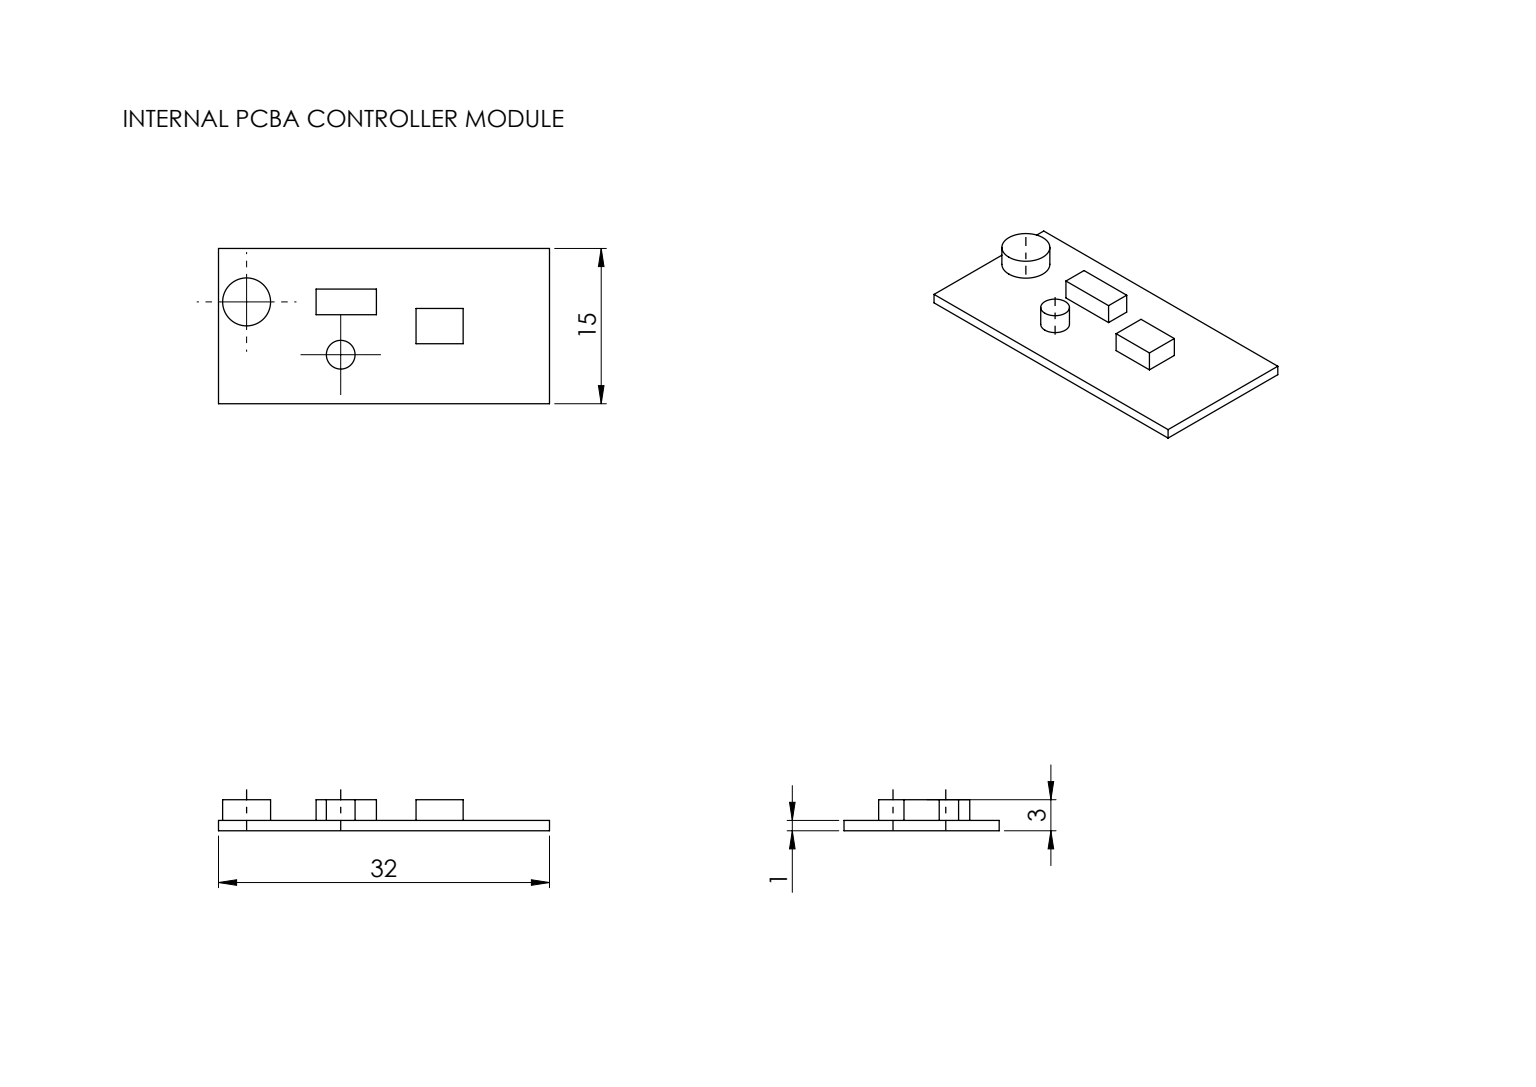
ISO-10303-21;
HEADER;
FILE_DESCRIPTION (('STEP AP214'),
    '1' );
FILE_NAME ('Internal PCBA Controller Module.step',
    '2026-10-02T09:26:43',
    ( '' ),
    ( '' ),
    'SwSTEP 2.0',
    'SolidWorks 2026',
    '' );
FILE_SCHEMA (( 'AUTOMOTIVE_DESIGN' ));
ENDSEC;

DATA;
#61=CARTESIAN_POINT ( 'NONE',  ( 139.9358549477330200, 0.5000000000000000000, -1.098523788719517169 ) ) ;
#111=CARTESIAN_POINT ( 'NONE',  ( 133.2169897921533845, 2.500000000000000000, -4.655597831175330548 ) ) ;
#208=FILL_AREA_STYLE ('',( #102307 ) ) ;
#396=PLANE ( 'NONE',  #56788 ) ;
#491=VECTOR ( 'NONE', #65782, 1000.000000000000000 ) ;
#598=DIRECTION ( 'NONE',  ( 0.000000000000000000, 0.000000000000000000, -1.000000000000000000 ) ) ;
#785=AXIS2_PLACEMENT_3D ( 'NONE', #25187, #6184, #3623 ) ;
#1353=DIRECTION ( 'NONE',  ( 1.000000000000000000, 0.000000000000000000, 0.000000000000000000 ) ) ;
#1618=AXIS2_PLACEMENT_3D ( 'NONE', #115980, #104231, #44031 ) ;
#1686=AXIS2_PLACEMENT_3D ( 'NONE', #69594, #89239, #129198 ) ;
#1783=ADVANCED_FACE ( 'NONE', ( #63659 ), #47886, .F. ) ;
#1952=LINE ( 'NONE', #55582, #72543 ) ;
#1992=EDGE_LOOP ( 'NONE', ( #83331, #6563, #5558, #78744 ) ) ;
#2013=VECTOR ( 'NONE', #33725, 1000.000000000000000 ) ;
#2082=CARTESIAN_POINT ( 'NONE',  ( 0.000000000000000000, 2.500000000000000000, 0.000000000000000000 ) ) ;
#2160=DIRECTION ( 'NONE',  ( 1.000000000000000000, 0.000000000000000000, 0.000000000000000000 ) ) ;
#2750=ORIENTED_EDGE ( 'NONE', *, *, #14810, .F. ) ;
#2868=VERTEX_POINT ( 'NONE', #9576 ) ;
#3123=FACE_BOUND ( 'NONE', #89319, .T. ) ;
#3196=DIRECTION ( 'NONE',  ( -0.000000000000000000, -1.000000000000000000, -0.000000000000000000 ) ) ;
#3623=DIRECTION ( 'NONE',  ( 0.000000000000000000, -0.000000000000000000, 1.000000000000000000 ) ) ;
#3643=ORIENTED_EDGE ( 'NONE', *, *, #119168, .T. ) ;
#3721=EDGE_LOOP ( 'NONE', ( #14930, #97877, #94219, #80001 ) ) ;
#3749=ADVANCED_FACE ( 'NONE', ( #85573 ), #33279, .F. ) ;
#4146=ORIENTED_EDGE ( 'NONE', *, *, #13081, .F. ) ;
#4176=VERTEX_POINT ( 'NONE', #110095 ) ;
#4584=DIRECTION ( 'NONE',  ( 0.000000000000000000, -0.000000000000000000, 1.000000000000000000 ) ) ;
#4890=CARTESIAN_POINT ( 'NONE',  ( 149.5981739382431783, 2.500000000000000000, 1.703575533167231537 ) ) ;
#5071=DIRECTION ( 'NONE',  ( 1.000000000000000000, 0.000000000000000000, -1.084202172485504434E-16 ) ) ;
#5285=CARTESIAN_POINT ( 'NONE',  ( 139.9358549477330200, 2.500000000000000000, -3.576063159858998475 ) ) ;
#5558=ORIENTED_EDGE ( 'NONE', *, *, #35698, .F. ) ;
#5707=CARTESIAN_POINT ( 'NONE',  ( 154.1524742528378056, 0.5000000000000000000, 1.703575533167231537 ) ) ;
#5990=SURFACE_SIDE_STYLE ('',( #85210 ) ) ;
#6007=CARTESIAN_POINT ( 'NONE',  ( 130.5000000000000000, -0.5000000000000000000, 7.499999999999998224 ) ) ;
#6184=DIRECTION ( 'NONE',  ( 0.000000000000000000, 1.000000000000000000, 0.000000000000000000 ) ) ;
#6305=AXIS2_PLACEMENT_3D ( 'NONE', #84477, #104735, #4584 ) ;
#6563=ORIENTED_EDGE ( 'NONE', *, *, #82060, .F. ) ;
#6883=EDGE_CURVE ( 'NONE', #54857, #102205, #70700, .T. ) ;
#6965=EDGE_LOOP ( 'NONE', ( #83440, #68214, #37688, #13118 ) ) ;
#7061=EDGE_LOOP ( 'NONE', ( #21290, #56050 ) ) ;
#7353=AXIS2_PLACEMENT_3D ( 'NONE', #115499, #75583, #67039 ) ;
#7874=FACE_OUTER_BOUND ( 'NONE', #93186, .T. ) ;
#8253=ORIENTED_EDGE ( 'NONE', *, *, #14810, .T. ) ;
#8378=AXIS2_PLACEMENT_3D ( 'NONE', #66138, #106073, #107999 ) ;
#8513=CARTESIAN_POINT ( 'NONE',  ( 162.5000000000000000, -0.5000000000000000000, -7.500000000000005329 ) ) ;
#9576=CARTESIAN_POINT ( 'NONE',  ( 142.3152275665817115, 0.5000000000000000000, 4.152444035927816302 ) ) ;
#9599=DIRECTION ( 'NONE',  ( -1.000000000000000000, -0.000000000000000000, -0.000000000000000000 ) ) ;
#9893=LINE ( 'NONE', #61, #77548 ) ;
#9916=AXIS2_PLACEMENT_3D ( 'NONE', #78615, #38022, #77944 ) ;
#9974=VECTOR ( 'NONE', #56454, 1000.000000000000000 ) ;
#10039=CARTESIAN_POINT ( 'NONE',  ( 162.5000000000000000, 0.5000000000000000000, -7.500000000000005329 ) ) ;
#10059=LINE ( 'NONE', #110195, #83855 ) ;
#10241=FACE_OUTER_BOUND ( 'NONE', #80105, .T. ) ;
#10407=ORIENTED_EDGE ( 'NONE', *, *, #13081, .T. ) ;
#10478=ORIENTED_EDGE ( 'NONE', *, *, #61124, .T. ) ;
#10519=EDGE_LOOP ( 'NONE', ( #14019, #2750, #22603, #90684 ) ) ;
#10639=VERTEX_POINT ( 'NONE', #6007 ) ;
#10644=CARTESIAN_POINT ( 'NONE',  ( 0.000000000000000000, 0.000000000000000000, 0.000000000000000000 ) ) ;
#10757=VECTOR ( 'NONE', #106512, 1000.000000000000000 ) ;
#10957=ORIENTED_EDGE ( 'NONE', *, *, #27576, .T. ) ;
#11366=CARTESIAN_POINT ( 'NONE',  ( 162.5000000000000000, 0.5000000000000000000, -7.500000000000005329 ) ) ;
#11835=CARTESIAN_POINT ( 'NONE',  ( 139.9358549477330200, 2.500000000000000000, -3.576063159858998475 ) ) ;
#11990=VERTEX_POINT ( 'NONE', #40618 ) ;
#12151=AXIS2_PLACEMENT_3D ( 'NONE', #80067, #19864, #119995 ) ;
#12406=ORIENTED_EDGE ( 'NONE', *, *, #65701, .T. ) ;
#12503=PLANE ( 'NONE',  #85742 ) ;
#12613=SURFACE_SIDE_STYLE ('',( #121939 ) ) ;
#12975=CARTESIAN_POINT ( 'NONE',  ( 142.3152275665817115, 2.500000000000000000, 4.152444035927816302 ) ) ;
#13081=EDGE_CURVE ( 'NONE', #86648, #112541, #57109, .T. ) ;
#13118=ORIENTED_EDGE ( 'NONE', *, *, #102486, .T. ) ;
#13186=DIRECTION ( 'NONE',  ( 0.000000000000000000, -0.000000000000000000, 1.000000000000000000 ) ) ;
#13431=VECTOR ( 'NONE', #66560, 1000.000000000000000 ) ;
#13502=CARTESIAN_POINT ( 'NONE',  ( 145.7653593504141725, 0.5000000000000000000, -3.576063159858998475 ) ) ;
#13560=AXIS2_PLACEMENT_3D ( 'NONE', #118011, #28360, #95800 ) ;
#13601=PLANE ( 'NONE',  #20802 ) ;
#13681=ORIENTED_EDGE ( 'NONE', *, *, #25639, .T. ) ;
#13709=DIRECTION ( 'NONE',  ( 0.000000000000000000, 0.000000000000000000, 1.000000000000000000 ) ) ;
#13884=SURFACE_STYLE_USAGE ( .BOTH. , #5990 ) ;
#13959=ORIENTED_EDGE ( 'NONE', *, *, #40890, .T. ) ;
#14019=ORIENTED_EDGE ( 'NONE', *, *, #43973, .T. ) ;
#14045=UNCERTAINTY_MEASURE_WITH_UNIT (LENGTH_MEASURE( 1.000000000000000082E-05 ), #22472, 'distance_accuracy_value', 'NONE');
#14204=DIRECTION ( 'NONE',  ( 0.000000000000000000, 1.000000000000000000, 0.000000000000000000 ) ) ;
#14467=CARTESIAN_POINT ( 'NONE',  ( 133.2169897921533845, 0.5000000000000000000, -0.01898911740318533561 ) ) ;
#14810=EDGE_CURVE ( 'NONE', #34747, #62008, #64855, .T. ) ;
#14860=DIRECTION ( 'NONE',  ( 0.000000000000000000, 0.000000000000000000, 1.000000000000000000 ) ) ;
#14930=ORIENTED_EDGE ( 'NONE', *, *, #99140, .F. ) ;
#15162=MECHANICAL_DESIGN_GEOMETRIC_PRESENTATION_REPRESENTATION('',(#56927),#17210);
#15699=EDGE_CURVE ( 'NONE', #104225, #83642, #112378, .T. ) ;
#16019=ADVANCED_FACE ( 'NONE', ( #91766 ), #92401, .T. ) ;
#16201=EDGE_LOOP ( 'NONE', ( #89223, #108455, #3643, #45452 ) ) ;
#16389=DIRECTION ( 'NONE',  ( -0.000000000000000000, -0.000000000000000000, -1.000000000000000000 ) ) ;
#16519=CARTESIAN_POINT ( 'NONE',  ( 133.2169897921533845, 2.500000000000000000, -4.655597831175330548 ) ) ;
#16562=LINE ( 'NONE', #104324, #48735 ) ;
#16982=CARTESIAN_POINT ( 'NONE',  ( 154.1524742528378056, 2.500000000000000000, -1.703575533167231537 ) ) ;
#17147=DIRECTION ( 'NONE',  ( -0.000000000000000000, -1.000000000000000000, -0.000000000000000000 ) ) ;
#17210=( GEOMETRIC_REPRESENTATION_CONTEXT ( 3 ) GLOBAL_UNCERTAINTY_ASSIGNED_CONTEXT ( ( #14045 ) ) GLOBAL_UNIT_ASSIGNED_CONTEXT ( ( #22472, #129212, #51921 ) ) REPRESENTATION_CONTEXT ( 'NONE', 'WORKASPACE' ) );
#17798=CARTESIAN_POINT ( 'NONE',  ( 149.5981739382431783, 0.5000000000000000000, -1.703575533167231537 ) ) ;
#17924=APPLICATION_CONTEXT ( 'automotive_design' ) ;
#18114=DIRECTION ( 'NONE',  ( 0.000000000000000000, 0.000000000000000000, -1.000000000000000000 ) ) ;
#18288=EDGE_CURVE ( 'NONE', #70042, #49008, #44429, .T. ) ;
#18424=VECTOR ( 'NONE', #41452, 1000.000000000000000 ) ;
#19326=ORIENTED_EDGE ( 'NONE', *, *, #40152, .F. ) ;
#19545=PLANE ( 'NONE',  #115654 ) ;
#19570=CARTESIAN_POINT ( 'NONE',  ( 149.5981739382431783, 2.500000000000000000, 1.703575533167231537 ) ) ;
#19670=ORIENTED_EDGE ( 'NONE', *, *, #40152, .T. ) ;
#19864=DIRECTION ( 'NONE',  ( -0.000000000000000000, -1.000000000000000000, -0.000000000000000000 ) ) ;
#19875=EDGE_CURVE ( 'NONE', #37705, #4176, #75349, .T. ) ;
#20589=ADVANCED_FACE ( 'NONE', ( #86567 ), #57111, .T. ) ;
#20689=CARTESIAN_POINT ( 'NONE',  ( 130.5000000000000000, 0.5000000000000000000, 7.499999999999998224 ) ) ;
#20802=AXIS2_PLACEMENT_3D ( 'NONE', #25349, #65927, #45666 ) ;
#20814=CARTESIAN_POINT ( 'NONE',  ( 162.5000000000000000, -0.5000000000000000000, 7.499999999999994671 ) ) ;
#21137=FACE_OUTER_BOUND ( 'NONE', #70487, .T. ) ;
#21244=CARTESIAN_POINT ( 'NONE',  ( 133.2169897921533845, 2.500000000000000000, -2.337293474289257933 ) ) ;
#21290=ORIENTED_EDGE ( 'NONE', *, *, #30432, .T. ) ;
#21819=SURFACE_STYLE_USAGE ( .BOTH. , #12613 ) ;
#22472=( LENGTH_UNIT ( ) NAMED_UNIT ( * ) SI_UNIT ( .MILLI., .METRE. ) );
#22564=ADVANCED_FACE ( 'NONE', ( #109202 ), #19545, .F. ) ;
#22603=ORIENTED_EDGE ( 'NONE', *, *, #65701, .F. ) ;
#23083=EDGE_CURVE ( 'NONE', #4176, #10639, #30528, .T. ) ;
#23103=EDGE_LOOP ( 'NONE', ( #36300, #59458 ) ) ;
#23423=DIRECTION ( 'NONE',  ( 1.084202172485504434E-16, -0.000000000000000000, 1.000000000000000000 ) ) ;
#23907=VECTOR ( 'NONE', #113347, 1000.000000000000000 ) ;
#24055=EDGE_LOOP ( 'NONE', ( #40407, #101634, #105706, #26760 ) ) ;
#24276=ADVANCED_FACE ( 'NONE', ( #10241 ), #396, .F. ) ;
#24693=DIRECTION ( 'NONE',  ( 0.000000000000000000, 0.000000000000000000, 1.000000000000000000 ) ) ;
#25029=CARTESIAN_POINT ( 'NONE',  ( 133.2169897921533845, 0.5000000000000000000, -4.655597831175330548 ) ) ;
#25187=CARTESIAN_POINT ( 'NONE',  ( 133.2169897921533845, 2.500000000000000000, -2.337293474289257933 ) ) ;
#25349=CARTESIAN_POINT ( 'NONE',  ( 139.9358549477330200, 2.500000000000000000, -3.576063159858998475 ) ) ;
#25358=AXIS2_PLACEMENT_3D ( 'NONE', #125675, #49091, #598 ) ;
#25639=EDGE_CURVE ( 'NONE', #44247, #77073, #59607, .T. ) ;
#26495=EDGE_CURVE ( 'NONE', #117877, #112541, #89210, .T. ) ;
#26601=LINE ( 'NONE', #66508, #87205 ) ;
#26760=ORIENTED_EDGE ( 'NONE', *, *, #92525, .T. ) ;
#26825=DIRECTION ( 'NONE',  ( 0.000000000000000000, -0.000000000000000000, 1.000000000000000000 ) ) ;
#26933=ORIENTED_EDGE ( 'NONE', *, *, #107201, .F. ) ;
#26948=DIRECTION ( 'NONE',  ( -1.000000000000000000, 0.000000000000000000, -0.000000000000000000 ) ) ;
#27283=CARTESIAN_POINT ( 'NONE',  ( 149.5981739382431783, 0.5000000000000000000, 1.703575533167231537 ) ) ;
#27500=DIRECTION ( 'NONE',  ( -0.000000000000000000, -1.000000000000000000, -0.000000000000000000 ) ) ;
#27576=EDGE_CURVE ( 'NONE', #86599, #110722, #33227, .T. ) ;
#28107=ORIENTED_EDGE ( 'NONE', *, *, #120172, .T. ) ;
#28360=DIRECTION ( 'NONE',  ( 0.000000000000000000, 1.000000000000000000, 0.000000000000000000 ) ) ;
#28585=CARTESIAN_POINT ( 'NONE',  ( 149.5981739382431783, 2.500000000000000000, -1.703575533167231537 ) ) ;
#28690=VERTEX_POINT ( 'NONE', #77802 ) ;
#29807=DIRECTION ( 'NONE',  ( 0.000000000000000000, 0.000000000000000000, -1.000000000000000000 ) ) ;
#29930=VECTOR ( 'NONE', #73992, 1000.000000000000000 ) ;
#30207=ORIENTED_EDGE ( 'NONE', *, *, #40786, .F. ) ;
#30325=EDGE_LOOP ( 'NONE', ( #77414, #45887, #65344, #115571 ) ) ;
#30432=EDGE_CURVE ( 'NONE', #86599, #28690, #57484, .T. ) ;
#30528=LINE ( 'NONE', #20689, #36456 ) ;
#30686=EDGE_LOOP ( 'NONE', ( #63549, #119398, #71516, #120626 ) ) ;
#31267=LINE ( 'NONE', #62658, #109837 ) ;
#31683=ORIENTED_EDGE ( 'NONE', *, *, #15699, .F. ) ;
#32674=AXIS2_PLACEMENT_3D ( 'NONE', #63607, #104169, #74707 ) ;
#32686=AXIS2_PLACEMENT_3D ( 'NONE', #33242, #82977, #92124 ) ;
#32743=PLANE ( 'NONE',  #40256 ) ;
#32771=DIRECTION ( 'NONE',  ( -0.000000000000000000, -0.000000000000000000, -1.000000000000000000 ) ) ;
#33184=EDGE_CURVE ( 'NONE', #50067, #54857, #10059, .T. ) ;
#33227=LINE ( 'NONE', #73132, #113990 ) ;
#33242=CARTESIAN_POINT ( 'NONE',  ( 0.000000000000000000, 0.5000000000000000000, 0.000000000000000000 ) ) ;
#33279=PLANE ( 'NONE',  #54019 ) ;
#33446=ADVANCED_FACE ( 'NONE', ( #115195 ), #45850, .F. ) ;
#33725=DIRECTION ( 'NONE',  ( 1.000000000000000000, 0.000000000000000000, 0.000000000000000000 ) ) ;
#33856=FACE_BOUND ( 'NONE', #23103, .T. ) ;
#33922=ORIENTED_EDGE ( 'NONE', *, *, #100074, .F. ) ;
#34197=( NAMED_UNIT ( * ) SI_UNIT ( $, .STERADIAN. ) SOLID_ANGLE_UNIT ( ) );
#34567=CARTESIAN_POINT ( 'NONE',  ( 162.5000000000000000, 0.5000000000000000000, -7.500000000000005329 ) ) ;
#34673=ORIENTED_EDGE ( 'NONE', *, *, #35638, .T. ) ;
#34747=VERTEX_POINT ( 'NONE', #113159 ) ;
#35072=ORIENTED_EDGE ( 'NONE', *, *, #107639, .F. ) ;
#35319=DIRECTION ( 'NONE',  ( 1.000000000000000000, -0.000000000000000000, -1.084202172485504434E-16 ) ) ;
#35388=AXIS2_PLACEMENT_3D ( 'NONE', #11366, #98444, #38931 ) ;
#35483=FILL_AREA_STYLE ('',( #66208 ) ) ;
#35638=EDGE_CURVE ( 'NONE', #70042, #119203, #86366, .T. ) ;
#35698=EDGE_CURVE ( 'NONE', #4176, #104225, #16562, .T. ) ;
#36203=CARTESIAN_POINT ( 'NONE',  ( 0.000000000000000000, -0.5000000000000000000, 0.000000000000000000 ) ) ;
#36216=AXIS2_PLACEMENT_3D ( 'NONE', #21244, #71642, #72931 ) ;
#36253=ORIENTED_EDGE ( 'NONE', *, *, #107201, .T. ) ;
#36300=ORIENTED_EDGE ( 'NONE', *, *, #61124, .F. ) ;
#36456=VECTOR ( 'NONE', #112293, 1000.000000000000000 ) ;
#36596=ORIENTED_EDGE ( 'NONE', *, *, #6883, .T. ) ;
#36663=PLANE ( 'NONE',  #77580 ) ;
#36815=ORIENTED_EDGE ( 'NONE', *, *, #116805, .T. ) ;
#37667=EDGE_LOOP ( 'NONE', ( #50089, #99755, #58404, #85578 ) ) ;
#37688=ORIENTED_EDGE ( 'NONE', *, *, #72322, .F. ) ;
#37705=VERTEX_POINT ( 'NONE', #101594 ) ;
#37972=FACE_OUTER_BOUND ( 'NONE', #16201, .T. ) ;
#38022=DIRECTION ( 'NONE',  ( 0.000000000000000000, 0.000000000000000000, -1.000000000000000000 ) ) ;
#38442=LINE ( 'NONE', #108438, #10757 ) ;
#38571=DIRECTION ( 'NONE',  ( -1.000000000000000000, 0.000000000000000000, 1.084202172485504434E-16 ) ) ;
#38931=DIRECTION ( 'NONE',  ( 0.000000000000000000, 0.000000000000000000, 1.000000000000000000 ) ) ;
#39634=EDGE_CURVE ( 'NONE', #83642, #37705, #1952, .T. ) ;
#39846=VERTEX_POINT ( 'NONE', #20814 ) ;
#40130=ADVANCED_FACE ( 'NONE', ( #21137 ), #120634, .T. ) ;
#40152=EDGE_CURVE ( 'NONE', #83642, #44247, #48678, .T. ) ;
#40242=EDGE_CURVE ( 'NONE', #2868, #110722, #58145, .T. ) ;
#40256=AXIS2_PLACEMENT_3D ( 'NONE', #51729, #13709, #101469 ) ;
#40287=ORIENTED_EDGE ( 'NONE', *, *, #114150, .T. ) ;
#40407=ORIENTED_EDGE ( 'NONE', *, *, #40786, .T. ) ;
#40618=CARTESIAN_POINT ( 'NONE',  ( 145.7653593504141725, 0.5000000000000000000, -3.576063159858998475 ) ) ;
#40626=CARTESIAN_POINT ( 'NONE',  ( 145.7653593504141725, 2.500000000000000000, -1.098523788719517169 ) ) ;
#40786=EDGE_CURVE ( 'NONE', #88966, #44639, #123061, .T. ) ;
#40890=EDGE_CURVE ( 'NONE', #124382, #117877, #56238, .T. ) ;
#40988=AXIS2_PLACEMENT_3D ( 'NONE', #106716, #27500, #125702 ) ;
#41452=DIRECTION ( 'NONE',  ( -0.000000000000000000, -1.000000000000000000, -0.000000000000000000 ) ) ;
#41855=CARTESIAN_POINT ( 'NONE',  ( 154.1524742528378056, 2.500000000000000000, 1.703575533167231537 ) ) ;
#42492=ORIENTED_EDGE ( 'NONE', *, *, #95835, .T. ) ;
#43073=PLANE ( 'NONE',  #32686 ) ;
#43181=VECTOR ( 'NONE', #74376, 1000.000000000000000 ) ;
#43237=VECTOR ( 'NONE', #69116, 1000.000000000000000 ) ;
#43499=CIRCLE ( 'NONE', #129200, 2.318304356886072615 ) ;
#43573=( GEOMETRIC_REPRESENTATION_CONTEXT ( 3 ) GLOBAL_UNCERTAINTY_ASSIGNED_CONTEXT ( ( #121523 ) ) GLOBAL_UNIT_ASSIGNED_CONTEXT ( ( #115286, #55749, #95689 ) ) REPRESENTATION_CONTEXT ( 'NONE', 'WORKASPACE' ) );
#43973=EDGE_CURVE ( 'NONE', #11990, #62008, #31267, .T. ) ;
#44015=( NAMED_UNIT ( * ) PLANE_ANGLE_UNIT ( ) SI_UNIT ( $, .RADIAN. ) );
#44031=DIRECTION ( 'NONE',  ( 0.000000000000000000, 0.000000000000000000, 1.000000000000000000 ) ) ;
#44169=FACE_OUTER_BOUND ( 'NONE', #116361, .T. ) ;
#44247=VERTEX_POINT ( 'NONE', #76336 ) ;
#44320=FACE_BOUND ( 'NONE', #30325, .T. ) ;
#44429=LINE ( 'NONE', #122999, #52762 ) ;
#44639=VERTEX_POINT ( 'NONE', #105480 ) ;
#44777=VECTOR ( 'NONE', #89682, 1000.000000000000000 ) ;
#45235=DIRECTION ( 'NONE',  ( -0.000000000000000000, -1.000000000000000000, -0.000000000000000000 ) ) ;
#45452=ORIENTED_EDGE ( 'NONE', *, *, #56592, .T. ) ;
#45454=EDGE_CURVE ( 'NONE', #37705, #77073, #26601, .T. ) ;
#45571=CARTESIAN_POINT ( 'NONE',  ( 149.5981739382431783, 2.500000000000000000, -1.703575533167231537 ) ) ;
#45666=DIRECTION ( 'NONE',  ( 0.000000000000000000, 0.000000000000000000, -1.000000000000000000 ) ) ;
#45850=PLANE ( 'NONE',  #25358 ) ;
#45887=ORIENTED_EDGE ( 'NONE', *, *, #121541, .F. ) ;
#46473=CARTESIAN_POINT ( 'NONE',  ( 149.5981739382431783, 0.5000000000000000000, 1.703575533167231537 ) ) ;
#46543=FACE_OUTER_BOUND ( 'NONE', #118945, .T. ) ;
#47036=CIRCLE ( 'NONE', #13560, 2.318304356886072615 ) ;
#47302=CARTESIAN_POINT ( 'NONE',  ( 149.5981739382431783, 2.500000000000000000, 1.703575533167231537 ) ) ;
#47791=ORIENTED_EDGE ( 'NONE', *, *, #67874, .F. ) ;
#47886=PLANE ( 'NONE',  #72691 ) ;
#48273=ORIENTED_EDGE ( 'NONE', *, *, #76882, .F. ) ;
#48395=ORIENTED_EDGE ( 'NONE', *, *, #56592, .F. ) ;
#48678=LINE ( 'NONE', #10039, #18424 ) ;
#48735=VECTOR ( 'NONE', #96415, 1000.000000000000000 ) ;
#49008=VERTEX_POINT ( 'NONE', #14467 ) ;
#49033=VERTEX_POINT ( 'NONE', #127515 ) ;
#49091=DIRECTION ( 'NONE',  ( 1.000000000000000000, 0.000000000000000000, 0.000000000000000000 ) ) ;
#49246=EDGE_LOOP ( 'NONE', ( #86440, #127359, #110430, #94128 ) ) ;
#49560=ORIENTED_EDGE ( 'NONE', *, *, #86041, .F. ) ;
#49832=COLOUR_RGB ( '', 0.31764706, 0.68627451, 0.89019608) ;
#49841=CARTESIAN_POINT ( 'NONE',  ( 162.5000000000000000, 0.5000000000000000000, 7.499999999999994671 ) ) ;
#50067=VERTEX_POINT ( 'NONE', #90481 ) ;
#50089=ORIENTED_EDGE ( 'NONE', *, *, #19875, .T. ) ;
#51459=ORIENTED_EDGE ( 'NONE', *, *, #56230, .F. ) ;
#51729=CARTESIAN_POINT ( 'NONE',  ( 149.5981739382431783, 2.500000000000000000, -1.703575533167231537 ) ) ;
#51890=VECTOR ( 'NONE', #17147, 1000.000000000000000 ) ;
#51921=( NAMED_UNIT ( * ) SI_UNIT ( $, .STERADIAN. ) SOLID_ANGLE_UNIT ( ) );
#52159=UNCERTAINTY_MEASURE_WITH_UNIT (LENGTH_MEASURE( 1.000000000000000082E-05 ), #103580, 'distance_accuracy_value', 'NONE');
#52762=VECTOR ( 'NONE', #102697, 1000.000000000000000 ) ;
#53084=DIRECTION ( 'NONE',  ( 0.000000000000000000, 0.000000000000000000, 1.000000000000000000 ) ) ;
#54019=AXIS2_PLACEMENT_3D ( 'NONE', #34567, #23423, #5071 ) ;
#54819=ORIENTED_EDGE ( 'NONE', *, *, #25639, .F. ) ;
#54857=VERTEX_POINT ( 'NONE', #74561 ) ;
#55281=ORIENTED_EDGE ( 'NONE', *, *, #26495, .F. ) ;
#55335=CARTESIAN_POINT ( 'NONE',  ( 154.1524742528378056, 2.500000000000000000, -1.703575533167231537 ) ) ;
#55424=AXIS2_PLACEMENT_3D ( 'NONE', #104256, #76086, #56430 ) ;
#55582=CARTESIAN_POINT ( 'NONE',  ( 162.5000000000000000, 0.5000000000000000000, -7.500000000000005329 ) ) ;
#55658=DIRECTION ( 'NONE',  ( -0.000000000000000000, -1.000000000000000000, -0.000000000000000000 ) ) ;
#55746=LINE ( 'NONE', #57022, #77152 ) ;
#55749=( NAMED_UNIT ( * ) PLANE_ANGLE_UNIT ( ) SI_UNIT ( $, .RADIAN. ) );
#55757=AXIS2_PLACEMENT_3D ( 'NONE', #96944, #116581, #57684 ) ;
#55901=PRODUCT_DEFINITION_CONTEXT ( 'detailed design', #83124, 'design' ) ;
#55938=DIRECTION ( 'NONE',  ( -0.000000000000000000, -1.000000000000000000, -0.000000000000000000 ) ) ;
#56050=ORIENTED_EDGE ( 'NONE', *, *, #99140, .T. ) ;
#56230=EDGE_CURVE ( 'NONE', #10639, #39846, #123661, .T. ) ;
#56238=LINE ( 'NONE', #126284, #56942 ) ;
#56430=DIRECTION ( 'NONE',  ( 0.000000000000000000, 0.000000000000000000, 1.000000000000000000 ) ) ;
#56454=DIRECTION ( 'NONE',  ( -0.000000000000000000, -1.000000000000000000, -0.000000000000000000 ) ) ;
#56460=DIRECTION ( 'NONE',  ( 0.000000000000000000, -0.000000000000000000, -1.000000000000000000 ) ) ;
#56546=ORIENTED_EDGE ( 'NONE', *, *, #6883, .F. ) ;
#56592=EDGE_CURVE ( 'NONE', #99284, #49008, #43499, .T. ) ;
#56788=AXIS2_PLACEMENT_3D ( 'NONE', #99916, #110368, #18114 ) ;
#56864=PRODUCT_CONTEXT ( 'NONE', #17924, 'mechanical' ) ;
#56927=STYLED_ITEM ( 'NONE', ( #60465 ), #57280 ) ;
#56942=VECTOR ( 'NONE', #57543, 1000.000000000000000 ) ;
#57022=CARTESIAN_POINT ( 'NONE',  ( 145.7653593504141725, 2.500000000000000000, -3.576063159858998475 ) ) ;
#57109=LINE ( 'NONE', #47302, #51890 ) ;
#57111=PLANE ( 'NONE',  #123787 ) ;
#57280=MANIFOLD_SOLID_BREP ( 'Boss-Extrude2', #89605 ) ;
#57484=CIRCLE ( 'NONE', #55424, 1.388921157871087386 ) ;
#57543=DIRECTION ( 'NONE',  ( -0.000000000000000000, -1.000000000000000000, -0.000000000000000000 ) ) ;
#57548=EDGE_LOOP ( 'NONE', ( #33922, #54819, #26933, #51459 ) ) ;
#57684=DIRECTION ( 'NONE',  ( 1.000000000000000000, 0.000000000000000000, -0.000000000000000000 ) ) ;
#57948=ORIENTED_EDGE ( 'NONE', *, *, #26495, .T. ) ;
#58145=CIRCLE ( 'NONE', #1686, 1.388921157871087386 ) ;
#58233=DIRECTION ( 'NONE',  ( 0.000000000000000000, 1.000000000000000000, 0.000000000000000000 ) ) ;
#58307=ADVANCED_FACE ( 'NONE', ( #114851 ), #114226, .T. ) ;
#58404=ORIENTED_EDGE ( 'NONE', *, *, #15699, .T. ) ;
#58989=DIRECTION ( 'NONE',  ( 0.000000000000000000, 0.000000000000000000, -1.000000000000000000 ) ) ;
#59138=ORIENTED_EDGE ( 'NONE', *, *, #121057, .T. ) ;
#59458=ORIENTED_EDGE ( 'NONE', *, *, #40242, .F. ) ;
#59607=LINE ( 'NONE', #117174, #44777 ) ;
#60143=DIRECTION ( 'NONE',  ( -1.084202172485504434E-16, 0.000000000000000000, -1.000000000000000000 ) ) ;
#60465=PRESENTATION_STYLE_ASSIGNMENT (( #21819 ) ) ;
#60833=EDGE_LOOP ( 'NONE', ( #99588, #34673 ) ) ;
#61124=EDGE_CURVE ( 'NONE', #110722, #2868, #89086, .T. ) ;
#61369=ORIENTED_EDGE ( 'NONE', *, *, #33184, .F. ) ;
#61627=FACE_OUTER_BOUND ( 'NONE', #24055, .T. ) ;
#62008=VERTEX_POINT ( 'NONE', #72962 ) ;
#62280=CIRCLE ( 'NONE', #1618, 1.388921157871087386 ) ;
#62658=CARTESIAN_POINT ( 'NONE',  ( 139.9358549477330200, 0.5000000000000000000, -3.576063159858998475 ) ) ;
#63166=VECTOR ( 'NONE', #92728, 1000.000000000000000 ) ;
#63549=ORIENTED_EDGE ( 'NONE', *, *, #93014, .T. ) ;
#63573=CARTESIAN_POINT ( 'NONE',  ( 145.7653593504141725, 2.500000000000000000, -3.576063159858998475 ) ) ;
#63607=CARTESIAN_POINT ( 'NONE',  ( 142.3152275665817115, 0.5000000000000000000, 2.763522878056728693 ) ) ;
#63659=FACE_OUTER_BOUND ( 'NONE', #119127, .T. ) ;
#64518=VECTOR ( 'NONE', #55938, 1000.000000000000000 ) ;
#64634=LINE ( 'NONE', #104562, #83491 ) ;
#64855=LINE ( 'NONE', #5285, #124731 ) ;
#65273=VECTOR ( 'NONE', #32771, 1000.000000000000000 ) ;
#65344=ORIENTED_EDGE ( 'NONE', *, *, #121057, .F. ) ;
#65701=EDGE_CURVE ( 'NONE', #49033, #34747, #81861, .T. ) ;
#65736=DIRECTION ( 'NONE',  ( -1.000000000000000000, 0.000000000000000000, 0.000000000000000000 ) ) ;
#65782=DIRECTION ( 'NONE',  ( -0.000000000000000000, -0.000000000000000000, -1.000000000000000000 ) ) ;
#65890=CARTESIAN_POINT ( 'NONE',  ( 133.2169897921533845, 0.5000000000000000000, -2.337293474289257933 ) ) ;
#65927=DIRECTION ( 'NONE',  ( 1.000000000000000000, 0.000000000000000000, 0.000000000000000000 ) ) ;
#66038=DIRECTION ( 'NONE',  ( -1.000000000000000000, 0.000000000000000000, 1.084202172485504434E-16 ) ) ;
#66138=CARTESIAN_POINT ( 'NONE',  ( 133.2169897921533845, 2.500000000000000000, -2.337293474289257933 ) ) ;
#66208=FILL_AREA_STYLE_COLOUR ( '', #49832 ) ;
#66387=CARTESIAN_POINT ( 'NONE',  ( 145.7653593504141725, 2.500000000000000000, -3.576063159858998475 ) ) ;
#66508=CARTESIAN_POINT ( 'NONE',  ( 130.5000000000000000, 0.5000000000000000000, -7.500000000000001776 ) ) ;
#66523=STYLED_ITEM ( 'NONE', ( #95044 ), #122749 ) ;
#66560=DIRECTION ( 'NONE',  ( 1.000000000000000000, 0.000000000000000000, 0.000000000000000000 ) ) ;
#67039=DIRECTION ( 'NONE',  ( 0.000000000000000000, 0.000000000000000000, 1.000000000000000000 ) ) ;
#67874=EDGE_CURVE ( 'NONE', #124382, #86648, #117571, .T. ) ;
#68022=VECTOR ( 'NONE', #109498, 1000.000000000000000 ) ;
#68214=ORIENTED_EDGE ( 'NONE', *, *, #40890, .F. ) ;
#69116=DIRECTION ( 'NONE',  ( 0.000000000000000000, 0.000000000000000000, 1.000000000000000000 ) ) ;
#69449=DIRECTION ( 'NONE',  ( -0.000000000000000000, -1.000000000000000000, -0.000000000000000000 ) ) ;
#69594=CARTESIAN_POINT ( 'NONE',  ( 142.3152275665817115, 0.5000000000000000000, 2.763522878056728693 ) ) ;
#69644=PLANE ( 'NONE',  #35388 ) ;
#70042=VERTEX_POINT ( 'NONE', #92350 ) ;
#70487=EDGE_LOOP ( 'NONE', ( #78003, #123559, #42492, #73890 ) ) ;
#70700=LINE ( 'NONE', #40626, #86914 ) ;
#70895=ORIENTED_EDGE ( 'NONE', *, *, #30432, .F. ) ;
#71516=ORIENTED_EDGE ( 'NONE', *, *, #67874, .T. ) ;
#71642=DIRECTION ( 'NONE',  ( 0.000000000000000000, 1.000000000000000000, 0.000000000000000000 ) ) ;
#72322=EDGE_CURVE ( 'NONE', #129134, #124382, #74699, .T. ) ;
#72543=VECTOR ( 'NONE', #66038, 1000.000000000000000 ) ;
#72691=AXIS2_PLACEMENT_3D ( 'NONE', #127089, #58989, #26948 ) ;
#72765=DIRECTION ( 'NONE',  ( -1.000000000000000000, -0.000000000000000000, -0.000000000000000000 ) ) ;
#72931=DIRECTION ( 'NONE',  ( 0.000000000000000000, 0.000000000000000000, 1.000000000000000000 ) ) ;
#72962=CARTESIAN_POINT ( 'NONE',  ( 139.9358549477330200, 0.5000000000000000000, -3.576063159858998475 ) ) ;
#73132=CARTESIAN_POINT ( 'NONE',  ( 142.3152275665817115, 2.500000000000000000, 1.374601720185641973 ) ) ;
#73890=ORIENTED_EDGE ( 'NONE', *, *, #119168, .F. ) ;
#73992=DIRECTION ( 'NONE',  ( -1.000000000000000000, -0.000000000000000000, -0.000000000000000000 ) ) ;
#74254=AXIS2_PLACEMENT_3D ( 'NONE', #89375, #119456, #29807 ) ;
#74376=DIRECTION ( 'NONE',  ( -0.000000000000000000, -0.000000000000000000, -1.000000000000000000 ) ) ;
#74561=CARTESIAN_POINT ( 'NONE',  ( 145.7653593504141725, 2.500000000000000000, -1.098523788719517169 ) ) ;
#74699=LINE ( 'NONE', #113325, #108637 ) ;
#74707=DIRECTION ( 'NONE',  ( 0.000000000000000000, 0.000000000000000000, 1.000000000000000000 ) ) ;
#75349=LINE ( 'NONE', #106110, #23907 ) ;
#75574=CARTESIAN_POINT ( 'NONE',  ( 139.9358549477330200, 2.500000000000000000, -1.098523788719517169 ) ) ;
#75583=DIRECTION ( 'NONE',  ( 0.000000000000000000, 1.000000000000000000, 0.000000000000000000 ) ) ;
#75737=VECTOR ( 'NONE', #83835, 1000.000000000000000 ) ;
#76043=SHAPE_REPRESENTATION_RELATIONSHIP ( 'NONE' , 'NONE' ,  #125483, #122749 ) ;
#76086=DIRECTION ( 'NONE',  ( 0.000000000000000000, 1.000000000000000000, 0.000000000000000000 ) ) ;
#76336=CARTESIAN_POINT ( 'NONE',  ( 162.5000000000000000, -0.5000000000000000000, -7.500000000000005329 ) ) ;
#76522=ADVANCED_FACE ( 'NONE', ( #61627 ), #12503, .F. ) ;
#76530=ORIENTED_EDGE ( 'NONE', *, *, #86293, .F. ) ;
#76587=FACE_OUTER_BOUND ( 'NONE', #30686, .T. ) ;
#76625=ADVANCED_FACE ( 'NONE', ( #76587 ), #95587, .T. ) ;
#76882=EDGE_CURVE ( 'NONE', #28690, #2868, #81730, .T. ) ;
#77073=VERTEX_POINT ( 'NONE', #96065 ) ;
#77152=VECTOR ( 'NONE', #126435, 1000.000000000000000 ) ;
#77175=SHAPE_DEFINITION_REPRESENTATION ( #87007, #125483 ) ;
#77414=ORIENTED_EDGE ( 'NONE', *, *, #114150, .F. ) ;
#77548=VECTOR ( 'NONE', #1353, 1000.000000000000000 ) ;
#77580=AXIS2_PLACEMENT_3D ( 'NONE', #116474, #58233, #26825 ) ;
#77694=PRODUCT_DEFINITION_FORMATION_WITH_SPECIFIED_SOURCE ( 'ANY', '', #95331, .NOT_KNOWN. ) ;
#77802=CARTESIAN_POINT ( 'NONE',  ( 142.3152275665817115, 2.500000000000000000, 4.152444035927816302 ) ) ;
#77824=EDGE_CURVE ( 'NONE', #49033, #11990, #99791, .T. ) ;
#77944=DIRECTION ( 'NONE',  ( -1.000000000000000000, 0.000000000000000000, -0.000000000000000000 ) ) ;
#78003=ORIENTED_EDGE ( 'NONE', *, *, #35638, .F. ) ;
#78111=CARTESIAN_POINT ( 'NONE',  ( 149.5981739382431783, 0.5000000000000000000, -1.703575533167231537 ) ) ;
#78279=FACE_OUTER_BOUND ( 'NONE', #3721, .T. ) ;
#78325=LINE ( 'NONE', #129367, #100454 ) ;
#78615=CARTESIAN_POINT ( 'NONE',  ( 139.9358549477330200, 2.500000000000000000, -1.098523788719517169 ) ) ;
#78744=ORIENTED_EDGE ( 'NONE', *, *, #23083, .T. ) ;
#79265=ORIENTED_EDGE ( 'NONE', *, *, #120172, .F. ) ;
#79592=LINE ( 'NONE', #98555, #43237 ) ;
#80001=ORIENTED_EDGE ( 'NONE', *, *, #27576, .F. ) ;
#80067=CARTESIAN_POINT ( 'NONE',  ( 133.2169897921533845, 2.500000000000000000, -2.337293474289257933 ) ) ;
#80105=EDGE_LOOP ( 'NONE', ( #57948, #4146, #47791, #13959 ) ) ;
#80157=EDGE_LOOP ( 'NONE', ( #48395, #89825 ) ) ;
#80365=DIRECTION ( 'NONE',  ( -1.000000000000000000, -0.000000000000000000, -0.000000000000000000 ) ) ;
#80718=DIRECTION ( 'NONE',  ( 1.000000000000000000, 0.000000000000000000, 0.000000000000000000 ) ) ;
#81668=FACE_OUTER_BOUND ( 'NONE', #37667, .T. ) ;
#81730=LINE ( 'NONE', #12975, #96295 ) ;
#81861=LINE ( 'NONE', #11835, #29930 ) ;
#81876=DIRECTION ( 'NONE',  ( -1.000000000000000000, 0.000000000000000000, 0.000000000000000000 ) ) ;
#81932=DIRECTION ( 'NONE',  ( 0.000000000000000000, 1.000000000000000000, 0.000000000000000000 ) ) ;
#82060=EDGE_CURVE ( 'NONE', #104225, #39846, #96988, .T. ) ;
#82977=DIRECTION ( 'NONE',  ( 0.000000000000000000, -1.000000000000000000, 0.000000000000000000 ) ) ;
#83041=ORIENTED_EDGE ( 'NONE', *, *, #92525, .F. ) ;
#83124=APPLICATION_CONTEXT ( 'automotive_design' ) ;
#83181=MECHANICAL_DESIGN_GEOMETRIC_PRESENTATION_REPRESENTATION('',(#66523),#43573);
#83331=ORIENTED_EDGE ( 'NONE', *, *, #56230, .T. ) ;
#83440=ORIENTED_EDGE ( 'NONE', *, *, #107639, .T. ) ;
#83491=VECTOR ( 'NONE', #14860, 1000.000000000000000 ) ;
#83636=ADVANCED_FACE ( 'NONE', ( #117205 ), #118518, .F. ) ;
#83642=VERTEX_POINT ( 'NONE', #98234 ) ;
#83835=DIRECTION ( 'NONE',  ( -0.000000000000000000, -1.000000000000000000, -0.000000000000000000 ) ) ;
#83855=VECTOR ( 'NONE', #2160, 1000.000000000000000 ) ;
#83951=VECTOR ( 'NONE', #9599, 1000.000000000000000 ) ;
#84477=CARTESIAN_POINT ( 'NONE',  ( 0.000000000000000000, 2.500000000000000000, 0.000000000000000000 ) ) ;
#85036=ORIENTED_EDGE ( 'NONE', *, *, #86293, .T. ) ;
#85210=SURFACE_STYLE_FILL_AREA ( #35483 ) ;
#85573=FACE_OUTER_BOUND ( 'NONE', #98567, .T. ) ;
#85578=ORIENTED_EDGE ( 'NONE', *, *, #39634, .T. ) ;
#85742=AXIS2_PLACEMENT_3D ( 'NONE', #123730, #81876, #53084 ) ;
#86041=EDGE_CURVE ( 'NONE', #86648, #110490, #92645, .T. ) ;
#86293=EDGE_CURVE ( 'NONE', #50067, #120204, #116145, .T. ) ;
#86366=CIRCLE ( 'NONE', #36216, 2.318304356886072615 ) ;
#86374=FACE_OUTER_BOUND ( 'NONE', #7061, .T. ) ;
#86440=ORIENTED_EDGE ( 'NONE', *, *, #100074, .T. ) ;
#86561=LINE ( 'NONE', #16519, #9974 ) ;
#86567=FACE_OUTER_BOUND ( 'NONE', #57548, .T. ) ;
#86599=VERTEX_POINT ( 'NONE', #115162 ) ;
#86648=VERTEX_POINT ( 'NONE', #19570 ) ;
#86914=VECTOR ( 'NONE', #99533, 1000.000000000000000 ) ;
#86949=ADVANCED_FACE ( 'NONE', ( #103295 ), #13601, .F. ) ;
#87007=PRODUCT_DEFINITION_SHAPE ( 'NONE', 'NONE',  #92424 ) ;
#87205=VECTOR ( 'NONE', #106442, 1000.000000000000000 ) ;
#88416=CARTESIAN_POINT ( 'NONE',  ( 139.9358549477330200, 0.5000000000000000000, -1.098523788719517169 ) ) ;
#88966=VERTEX_POINT ( 'NONE', #5707 ) ;
#89086=CIRCLE ( 'NONE', #32674, 1.388921157871087386 ) ;
#89210=LINE ( 'NONE', #78111, #68022 ) ;
#89223=ORIENTED_EDGE ( 'NONE', *, *, #18288, .F. ) ;
#89239=DIRECTION ( 'NONE',  ( 0.000000000000000000, 1.000000000000000000, 0.000000000000000000 ) ) ;
#89319=EDGE_LOOP ( 'NONE', ( #30207, #125882, #55281, #35072 ) ) ;
#89373=AXIS2_PLACEMENT_3D ( 'NONE', #66387, #65736, #106315 ) ;
#89375=CARTESIAN_POINT ( 'NONE',  ( 142.3152275665817115, 2.500000000000000000, 2.763522878056728693 ) ) ;
#89587=ADVANCED_FACE ( 'NONE', ( #89921 ), #69644, .F. ) ;
#89605=CLOSED_SHELL ( 'NONE', ( #40130, #128218, #98175, #33446, #22564, #89587, #3749, #20589, #98751, #83636, #86949, #129142, #16019, #111605, #92078, #113651, #58307, #76522, #126752, #24276, #1783, #76625 ) ) ;
#89682=DIRECTION ( 'NONE',  ( -1.000000000000000000, 0.000000000000000000, 1.084202172485504434E-16 ) ) ;
#89825=ORIENTED_EDGE ( 'NONE', *, *, #95835, .F. ) ;
#89921=FACE_OUTER_BOUND ( 'NONE', #91344, .T. ) ;
#90481=CARTESIAN_POINT ( 'NONE',  ( 139.9358549477330200, 2.500000000000000000, -1.098523788719517169 ) ) ;
#90516=DIRECTION ( 'NONE',  ( 0.000000000000000000, 0.000000000000000000, 1.000000000000000000 ) ) ;
#90684=ORIENTED_EDGE ( 'NONE', *, *, #77824, .T. ) ;
#91344=EDGE_LOOP ( 'NONE', ( #36253, #19326, #31683, #125416 ) ) ;
#91640=FACE_OUTER_BOUND ( 'NONE', #6965, .T. ) ;
#91766=FACE_OUTER_BOUND ( 'NONE', #120854, .T. ) ;
#92025=LINE ( 'NONE', #120842, #83951 ) ;
#92078=ADVANCED_FACE ( 'NONE', ( #86374 ), #36663, .T. ) ;
#92124=DIRECTION ( 'NONE',  ( 0.000000000000000000, -0.000000000000000000, -1.000000000000000000 ) ) ;
#92350=CARTESIAN_POINT ( 'NONE',  ( 133.2169897921533845, 2.500000000000000000, -0.01898911740318533561 ) ) ;
#92401=PLANE ( 'NONE',  #129051 ) ;
#92424=PRODUCT_DEFINITION ( 'UNKNOWN', '', #77694, #55901 ) ;
#92525=EDGE_CURVE ( 'NONE', #110490, #88966, #38442, .T. ) ;
#92645=LINE ( 'NONE', #4890, #2013 ) ;
#92728=DIRECTION ( 'NONE',  ( -0.000000000000000000, -0.000000000000000000, -1.000000000000000000 ) ) ;
#92877=VECTOR ( 'NONE', #69449, 1000.000000000000000 ) ;
#93014=EDGE_CURVE ( 'NONE', #110490, #129134, #125354, .T. ) ;
#93186=EDGE_LOOP ( 'NONE', ( #48273, #70895, #10957, #10478 ) ) ;
#93371=LINE ( 'NONE', #13502, #63166 ) ;
#94128=ORIENTED_EDGE ( 'NONE', *, *, #45454, .T. ) ;
#94219=ORIENTED_EDGE ( 'NONE', *, *, #40242, .T. ) ;
#94275=ORIENTED_EDGE ( 'NONE', *, *, #98526, .T. ) ;
#95044=PRESENTATION_STYLE_ASSIGNMENT (( #13884 ) ) ;
#95331=PRODUCT ( 'Internal PCBA Controller Module', 'Internal PCBA Controller Module', '', ( #56864 ) ) ;
#95587=PLANE ( 'NONE',  #6305 ) ;
#95625=CYLINDRICAL_SURFACE ( 'NONE', #40988, 1.388921157871086942 ) ;
#95689=( NAMED_UNIT ( * ) SI_UNIT ( $, .STERADIAN. ) SOLID_ANGLE_UNIT ( ) );
#95800=DIRECTION ( 'NONE',  ( 0.000000000000000000, 0.000000000000000000, 1.000000000000000000 ) ) ;
#95835=EDGE_CURVE ( 'NONE', #49008, #99284, #47036, .T. ) ;
#96065=CARTESIAN_POINT ( 'NONE',  ( 130.5000000000000000, -0.5000000000000000000, -7.500000000000001776 ) ) ;
#96134=ORIENTED_EDGE ( 'NONE', *, *, #77824, .F. ) ;
#96234=CYLINDRICAL_SURFACE ( 'NONE', #8378, 2.318304356886073059 ) ;
#96295=VECTOR ( 'NONE', #3196, 1000.000000000000000 ) ;
#96415=DIRECTION ( 'NONE',  ( 1.000000000000000000, -0.000000000000000000, -1.084202172485504434E-16 ) ) ;
#96722=CARTESIAN_POINT ( 'NONE',  ( 142.3152275665817115, 0.5000000000000000000, 1.374601720185641973 ) ) ;
#96944=CARTESIAN_POINT ( 'NONE',  ( 139.9358549477330200, 2.500000000000000000, -3.576063159858998475 ) ) ;
#96988=LINE ( 'NONE', #49841, #92877 ) ;
#97877=ORIENTED_EDGE ( 'NONE', *, *, #76882, .T. ) ;
#98175=ADVANCED_FACE ( 'NONE', ( #123518, #33856, #44320, #81668, #3123 ), #43073, .F. ) ;
#98234=CARTESIAN_POINT ( 'NONE',  ( 162.5000000000000000, 0.5000000000000000000, -7.500000000000005329 ) ) ;
#98444=DIRECTION ( 'NONE',  ( -1.000000000000000000, 0.000000000000000000, 0.000000000000000000 ) ) ;
#98526=EDGE_CURVE ( 'NONE', #34747, #50067, #79592, .T. ) ;
#98555=CARTESIAN_POINT ( 'NONE',  ( 139.9358549477330200, 2.500000000000000000, -3.576063159858998475 ) ) ;
#98561=DIRECTION ( 'NONE',  ( 0.000000000000000000, 0.000000000000000000, 1.000000000000000000 ) ) ;
#98567=EDGE_LOOP ( 'NONE', ( #13681, #114723, #121173, #19670 ) ) ;
#98751=ADVANCED_FACE ( 'NONE', ( #44169 ), #115460, .F. ) ;
#99140=EDGE_CURVE ( 'NONE', #28690, #86599, #62280, .T. ) ;
#99284=VERTEX_POINT ( 'NONE', #25029 ) ;
#99533=DIRECTION ( 'NONE',  ( -0.000000000000000000, -1.000000000000000000, -0.000000000000000000 ) ) ;
#99588=ORIENTED_EDGE ( 'NONE', *, *, #117257, .T. ) ;
#99755=ORIENTED_EDGE ( 'NONE', *, *, #35698, .T. ) ;
#99791=LINE ( 'NONE', #63573, #75737 ) ;
#99916=CARTESIAN_POINT ( 'NONE',  ( 149.5981739382431783, 2.500000000000000000, -1.703575533167231537 ) ) ;
#100074=EDGE_CURVE ( 'NONE', #77073, #10639, #64634, .T. ) ;
#100454=VECTOR ( 'NONE', #98561, 1000.000000000000000 ) ;
#101469=DIRECTION ( 'NONE',  ( 1.000000000000000000, 0.000000000000000000, -0.000000000000000000 ) ) ;
#101594=CARTESIAN_POINT ( 'NONE',  ( 130.5000000000000000, 0.5000000000000000000, -7.500000000000001776 ) ) ;
#101634=ORIENTED_EDGE ( 'NONE', *, *, #102486, .F. ) ;
#102205=VERTEX_POINT ( 'NONE', #113285 ) ;
#102307=FILL_AREA_STYLE_COLOUR ( '', #102920 ) ;
#102486=EDGE_CURVE ( 'NONE', #129134, #44639, #126344, .T. ) ;
#102697=DIRECTION ( 'NONE',  ( -0.000000000000000000, -1.000000000000000000, -0.000000000000000000 ) ) ;
#102920=COLOUR_RGB ( '', 0.31764706, 0.68627451, 0.89019608) ;
#103295=FACE_OUTER_BOUND ( 'NONE', #114993, .T. ) ;
#103512=ORIENTED_EDGE ( 'NONE', *, *, #98526, .F. ) ;
#103580=( LENGTH_UNIT ( ) NAMED_UNIT ( * ) SI_UNIT ( .MILLI., .METRE. ) );
#104169=DIRECTION ( 'NONE',  ( 0.000000000000000000, 1.000000000000000000, 0.000000000000000000 ) ) ;
#104225=VERTEX_POINT ( 'NONE', #120382 ) ;
#104231=DIRECTION ( 'NONE',  ( 0.000000000000000000, 1.000000000000000000, 0.000000000000000000 ) ) ;
#104256=CARTESIAN_POINT ( 'NONE',  ( 142.3152275665817115, 2.500000000000000000, 2.763522878056728693 ) ) ;
#104324=CARTESIAN_POINT ( 'NONE',  ( 162.5000000000000000, 0.5000000000000000000, 7.499999999999994671 ) ) ;
#104562=CARTESIAN_POINT ( 'NONE',  ( 130.5000000000000000, -0.5000000000000000000, -7.500000000000001776 ) ) ;
#104735=DIRECTION ( 'NONE',  ( 0.000000000000000000, 1.000000000000000000, 0.000000000000000000 ) ) ;
#105065=VECTOR ( 'NONE', #16389, 1000.000000000000000 ) ;
#105480=CARTESIAN_POINT ( 'NONE',  ( 154.1524742528378056, 0.5000000000000000000, -1.703575533167231537 ) ) ;
#105706=ORIENTED_EDGE ( 'NONE', *, *, #93014, .F. ) ;
#106073=DIRECTION ( 'NONE',  ( -0.000000000000000000, -1.000000000000000000, -0.000000000000000000 ) ) ;
#106092=LINE ( 'NONE', #8513, #105065 ) ;
#106110=CARTESIAN_POINT ( 'NONE',  ( 130.5000000000000000, 0.5000000000000000000, -7.500000000000001776 ) ) ;
#106243=( GEOMETRIC_REPRESENTATION_CONTEXT ( 3 ) GLOBAL_UNCERTAINTY_ASSIGNED_CONTEXT ( ( #52159 ) ) GLOBAL_UNIT_ASSIGNED_CONTEXT ( ( #103580, #44015, #34197 ) ) REPRESENTATION_CONTEXT ( 'NONE', 'WORKASPACE' ) );
#106315=DIRECTION ( 'NONE',  ( 0.000000000000000000, 0.000000000000000000, 1.000000000000000000 ) ) ;
#106442=DIRECTION ( 'NONE',  ( -0.000000000000000000, -1.000000000000000000, -0.000000000000000000 ) ) ;
#106512=DIRECTION ( 'NONE',  ( -0.000000000000000000, -1.000000000000000000, -0.000000000000000000 ) ) ;
#106716=CARTESIAN_POINT ( 'NONE',  ( 142.3152275665817115, 2.500000000000000000, 2.763522878056728693 ) ) ;
#107123=DIRECTION ( 'NONE',  ( 0.000000000000000000, 0.000000000000000000, 1.000000000000000000 ) ) ;
#107201=EDGE_CURVE ( 'NONE', #39846, #44247, #106092, .T. ) ;
#107639=EDGE_CURVE ( 'NONE', #44639, #117877, #92025, .T. ) ;
#107999=DIRECTION ( 'NONE',  ( 0.000000000000000000, 0.000000000000000000, -1.000000000000000000 ) ) ;
#108296=AXIS2_PLACEMENT_3D ( 'NONE', #10644, #90516, #80718 ) ;
#108438=CARTESIAN_POINT ( 'NONE',  ( 154.1524742528378056, 2.500000000000000000, 1.703575533167231537 ) ) ;
#108455=ORIENTED_EDGE ( 'NONE', *, *, #117257, .F. ) ;
#108637=VECTOR ( 'NONE', #72765, 1000.000000000000000 ) ;
#109202=FACE_OUTER_BOUND ( 'NONE', #1992, .T. ) ;
#109498=DIRECTION ( 'NONE',  ( 0.000000000000000000, 0.000000000000000000, 1.000000000000000000 ) ) ;
#109837=VECTOR ( 'NONE', #80365, 1000.000000000000000 ) ;
#110095=CARTESIAN_POINT ( 'NONE',  ( 130.5000000000000000, 0.5000000000000000000, 7.499999999999998224 ) ) ;
#110195=CARTESIAN_POINT ( 'NONE',  ( 139.9358549477330200, 2.500000000000000000, -1.098523788719517169 ) ) ;
#110368=DIRECTION ( 'NONE',  ( 1.000000000000000000, 0.000000000000000000, 0.000000000000000000 ) ) ;
#110430=ORIENTED_EDGE ( 'NONE', *, *, #19875, .F. ) ;
#110490=VERTEX_POINT ( 'NONE', #41855 ) ;
#110722=VERTEX_POINT ( 'NONE', #96722 ) ;
#111605=ADVANCED_FACE ( 'NONE', ( #7874 ), #95625, .T. ) ;
#111839=CIRCLE ( 'NONE', #7353, 2.318304356886072615 ) ;
#112293=DIRECTION ( 'NONE',  ( -0.000000000000000000, -1.000000000000000000, -0.000000000000000000 ) ) ;
#112378=LINE ( 'NONE', #114929, #43181 ) ;
#112541=VERTEX_POINT ( 'NONE', #46473 ) ;
#113046=DIRECTION ( 'NONE',  ( -0.000000000000000000, -1.000000000000000000, -0.000000000000000000 ) ) ;
#113159=CARTESIAN_POINT ( 'NONE',  ( 139.9358549477330200, 2.500000000000000000, -3.576063159858998475 ) ) ;
#113285=CARTESIAN_POINT ( 'NONE',  ( 145.7653593504141725, 0.5000000000000000000, -1.098523788719517169 ) ) ;
#113325=CARTESIAN_POINT ( 'NONE',  ( 149.5981739382431783, 2.500000000000000000, -1.703575533167231537 ) ) ;
#113347=DIRECTION ( 'NONE',  ( 0.000000000000000000, 0.000000000000000000, 1.000000000000000000 ) ) ;
#113651=ADVANCED_FACE ( 'NONE', ( #37972 ), #96234, .T. ) ;
#113887=CARTESIAN_POINT ( 'NONE',  ( 154.1524742528378056, 0.5000000000000000000, -1.703575533167231537 ) ) ;
#113990=VECTOR ( 'NONE', #113046, 1000.000000000000000 ) ;
#114150=EDGE_CURVE ( 'NONE', #102205, #11990, #93371, .T. ) ;
#114226=PLANE ( 'NONE',  #785 ) ;
#114306=VECTOR ( 'NONE', #35319, 1000.000000000000000 ) ;
#114375=LINE ( 'NONE', #27283, #13431 ) ;
#114723=ORIENTED_EDGE ( 'NONE', *, *, #45454, .F. ) ;
#114851=FACE_OUTER_BOUND ( 'NONE', #60833, .T. ) ;
#114929=CARTESIAN_POINT ( 'NONE',  ( 162.5000000000000000, 0.5000000000000000000, -7.500000000000005329 ) ) ;
#114993=EDGE_LOOP ( 'NONE', ( #59138, #76530, #103512, #8253 ) ) ;
#115162=CARTESIAN_POINT ( 'NONE',  ( 142.3152275665817115, 2.500000000000000000, 1.374601720185641973 ) ) ;
#115195=FACE_OUTER_BOUND ( 'NONE', #49246, .T. ) ;
#115286=( LENGTH_UNIT ( ) NAMED_UNIT ( * ) SI_UNIT ( .MILLI., .METRE. ) );
#115360=DIRECTION ( 'NONE',  ( 0.000000000000000000, -1.000000000000000000, 0.000000000000000000 ) ) ;
#115460=PLANE ( 'NONE',  #89373 ) ;
#115499=CARTESIAN_POINT ( 'NONE',  ( 133.2169897921533845, 2.500000000000000000, -2.337293474289257933 ) ) ;
#115571=ORIENTED_EDGE ( 'NONE', *, *, #43973, .F. ) ;
#115654=AXIS2_PLACEMENT_3D ( 'NONE', #120332, #60143, #38571 ) ;
#115980=CARTESIAN_POINT ( 'NONE',  ( 142.3152275665817115, 2.500000000000000000, 2.763522878056728693 ) ) ;
#116145=LINE ( 'NONE', #75574, #64518 ) ;
#116361=EDGE_LOOP ( 'NONE', ( #40287, #96134, #79265, #36596 ) ) ;
#116427=CARTESIAN_POINT ( 'NONE',  ( 162.5000000000000000, -0.5000000000000000000, 7.499999999999994671 ) ) ;
#116474=CARTESIAN_POINT ( 'NONE',  ( 142.3152275665817115, 2.500000000000000000, 2.763522878056728693 ) ) ;
#116581=DIRECTION ( 'NONE',  ( 0.000000000000000000, 0.000000000000000000, 1.000000000000000000 ) ) ;
#116805=EDGE_CURVE ( 'NONE', #112541, #88966, #114375, .T. ) ;
#117174=CARTESIAN_POINT ( 'NONE',  ( 162.5000000000000000, -0.5000000000000000000, -7.500000000000005329 ) ) ;
#117205=FACE_OUTER_BOUND ( 'NONE', #10519, .T. ) ;
#117257=EDGE_CURVE ( 'NONE', #119203, #70042, #111839, .T. ) ;
#117571=LINE ( 'NONE', #28585, #118098 ) ;
#117877=VERTEX_POINT ( 'NONE', #17798 ) ;
#118011=CARTESIAN_POINT ( 'NONE',  ( 133.2169897921533845, 0.5000000000000000000, -2.337293474289257933 ) ) ;
#118098=VECTOR ( 'NONE', #107123, 1000.000000000000000 ) ;
#118518=PLANE ( 'NONE',  #55757 ) ;
#118945=EDGE_LOOP ( 'NONE', ( #121090, #56546, #61369, #85036 ) ) ;
#119127=EDGE_LOOP ( 'NONE', ( #36815, #83041, #49560, #10407 ) ) ;
#119168=EDGE_CURVE ( 'NONE', #119203, #99284, #86561, .T. ) ;
#119203=VERTEX_POINT ( 'NONE', #111 ) ;
#119398=ORIENTED_EDGE ( 'NONE', *, *, #72322, .T. ) ;
#119456=DIRECTION ( 'NONE',  ( -0.000000000000000000, -1.000000000000000000, -0.000000000000000000 ) ) ;
#119995=DIRECTION ( 'NONE',  ( 0.000000000000000000, 0.000000000000000000, -1.000000000000000000 ) ) ;
#120122=CYLINDRICAL_SURFACE ( 'NONE', #74254, 1.388921157871086942 ) ;
#120172=EDGE_CURVE ( 'NONE', #54857, #49033, #55746, .T. ) ;
#120204=VERTEX_POINT ( 'NONE', #88416 ) ;
#120332=CARTESIAN_POINT ( 'NONE',  ( 162.5000000000000000, 0.5000000000000000000, 7.499999999999994671 ) ) ;
#120382=CARTESIAN_POINT ( 'NONE',  ( 162.5000000000000000, 0.5000000000000000000, 7.499999999999994671 ) ) ;
#120626=ORIENTED_EDGE ( 'NONE', *, *, #86041, .T. ) ;
#120634=CYLINDRICAL_SURFACE ( 'NONE', #12151, 2.318304356886073059 ) ;
#120842=CARTESIAN_POINT ( 'NONE',  ( 149.5981739382431783, 0.5000000000000000000, -1.703575533167231537 ) ) ;
#120854=EDGE_LOOP ( 'NONE', ( #28107, #12406, #94275, #129030 ) ) ;
#121057=EDGE_CURVE ( 'NONE', #62008, #120204, #78325, .T. ) ;
#121090=ORIENTED_EDGE ( 'NONE', *, *, #121541, .T. ) ;
#121173=ORIENTED_EDGE ( 'NONE', *, *, #39634, .F. ) ;
#121468=VECTOR ( 'NONE', #55658, 1000.000000000000000 ) ;
#121523=UNCERTAINTY_MEASURE_WITH_UNIT (LENGTH_MEASURE( 1.000000000000000082E-05 ), #115286, 'distance_accuracy_value', 'NONE');
#121541=EDGE_CURVE ( 'NONE', #120204, #102205, #9893, .T. ) ;
#121939=SURFACE_STYLE_FILL_AREA ( #208 ) ;
#122749=ADVANCED_BREP_SHAPE_REPRESENTATION ( '', ( #57280, #108296 ), #106243 ) ;
#122999=CARTESIAN_POINT ( 'NONE',  ( 133.2169897921533845, 2.500000000000000000, -0.01898911740318533561 ) ) ;
#123061=LINE ( 'NONE', #113887, #65273 ) ;
#123518=FACE_BOUND ( 'NONE', #80157, .T. ) ;
#123559=ORIENTED_EDGE ( 'NONE', *, *, #18288, .T. ) ;
#123661=LINE ( 'NONE', #116427, #114306 ) ;
#123730=CARTESIAN_POINT ( 'NONE',  ( 154.1524742528378056, 2.500000000000000000, -1.703575533167231537 ) ) ;
#123787=AXIS2_PLACEMENT_3D ( 'NONE', #36203, #115360, #56460 ) ;
#124382=VERTEX_POINT ( 'NONE', #45571 ) ;
#124731=VECTOR ( 'NONE', #45235, 1000.000000000000000 ) ;
#125354=LINE ( 'NONE', #55335, #491 ) ;
#125416=ORIENTED_EDGE ( 'NONE', *, *, #82060, .T. ) ;
#125483=SHAPE_REPRESENTATION ( 'Internal PCBA Controller Module', ( #108296 ), #106243 ) ;
#125675=CARTESIAN_POINT ( 'NONE',  ( 130.5000000000000000, 0.5000000000000000000, -7.500000000000001776 ) ) ;
#125702=DIRECTION ( 'NONE',  ( 0.000000000000000000, 0.000000000000000000, -1.000000000000000000 ) ) ;
#125882=ORIENTED_EDGE ( 'NONE', *, *, #116805, .F. ) ;
#126284=CARTESIAN_POINT ( 'NONE',  ( 149.5981739382431783, 2.500000000000000000, -1.703575533167231537 ) ) ;
#126344=LINE ( 'NONE', #16982, #121468 ) ;
#126435=DIRECTION ( 'NONE',  ( -0.000000000000000000, -0.000000000000000000, -1.000000000000000000 ) ) ;
#126752=ADVANCED_FACE ( 'NONE', ( #91640 ), #32743, .F. ) ;
#127089=CARTESIAN_POINT ( 'NONE',  ( 149.5981739382431783, 2.500000000000000000, 1.703575533167231537 ) ) ;
#127359=ORIENTED_EDGE ( 'NONE', *, *, #23083, .F. ) ;
#127515=CARTESIAN_POINT ( 'NONE',  ( 145.7653593504141725, 2.500000000000000000, -3.576063159858998475 ) ) ;
#127689=CARTESIAN_POINT ( 'NONE',  ( 154.1524742528378056, 2.500000000000000000, -1.703575533167231537 ) ) ;
#128218=ADVANCED_FACE ( 'NONE', ( #78279 ), #120122, .T. ) ;
#128364=PLANE ( 'NONE',  #9916 ) ;
#129030=ORIENTED_EDGE ( 'NONE', *, *, #33184, .T. ) ;
#129051=AXIS2_PLACEMENT_3D ( 'NONE', #2082, #81932, #13186 ) ;
#129134=VERTEX_POINT ( 'NONE', #127689 ) ;
#129142=ADVANCED_FACE ( 'NONE', ( #46543 ), #128364, .F. ) ;
#129198=DIRECTION ( 'NONE',  ( 0.000000000000000000, 0.000000000000000000, 1.000000000000000000 ) ) ;
#129200=AXIS2_PLACEMENT_3D ( 'NONE', #65890, #14204, #24693 ) ;
#129212=( NAMED_UNIT ( * ) PLANE_ANGLE_UNIT ( ) SI_UNIT ( $, .RADIAN. ) );
#129367=CARTESIAN_POINT ( 'NONE',  ( 139.9358549477330200, 0.5000000000000000000, -3.576063159858998475 ) ) ;
ENDSEC;
END-ISO-10303-21;
